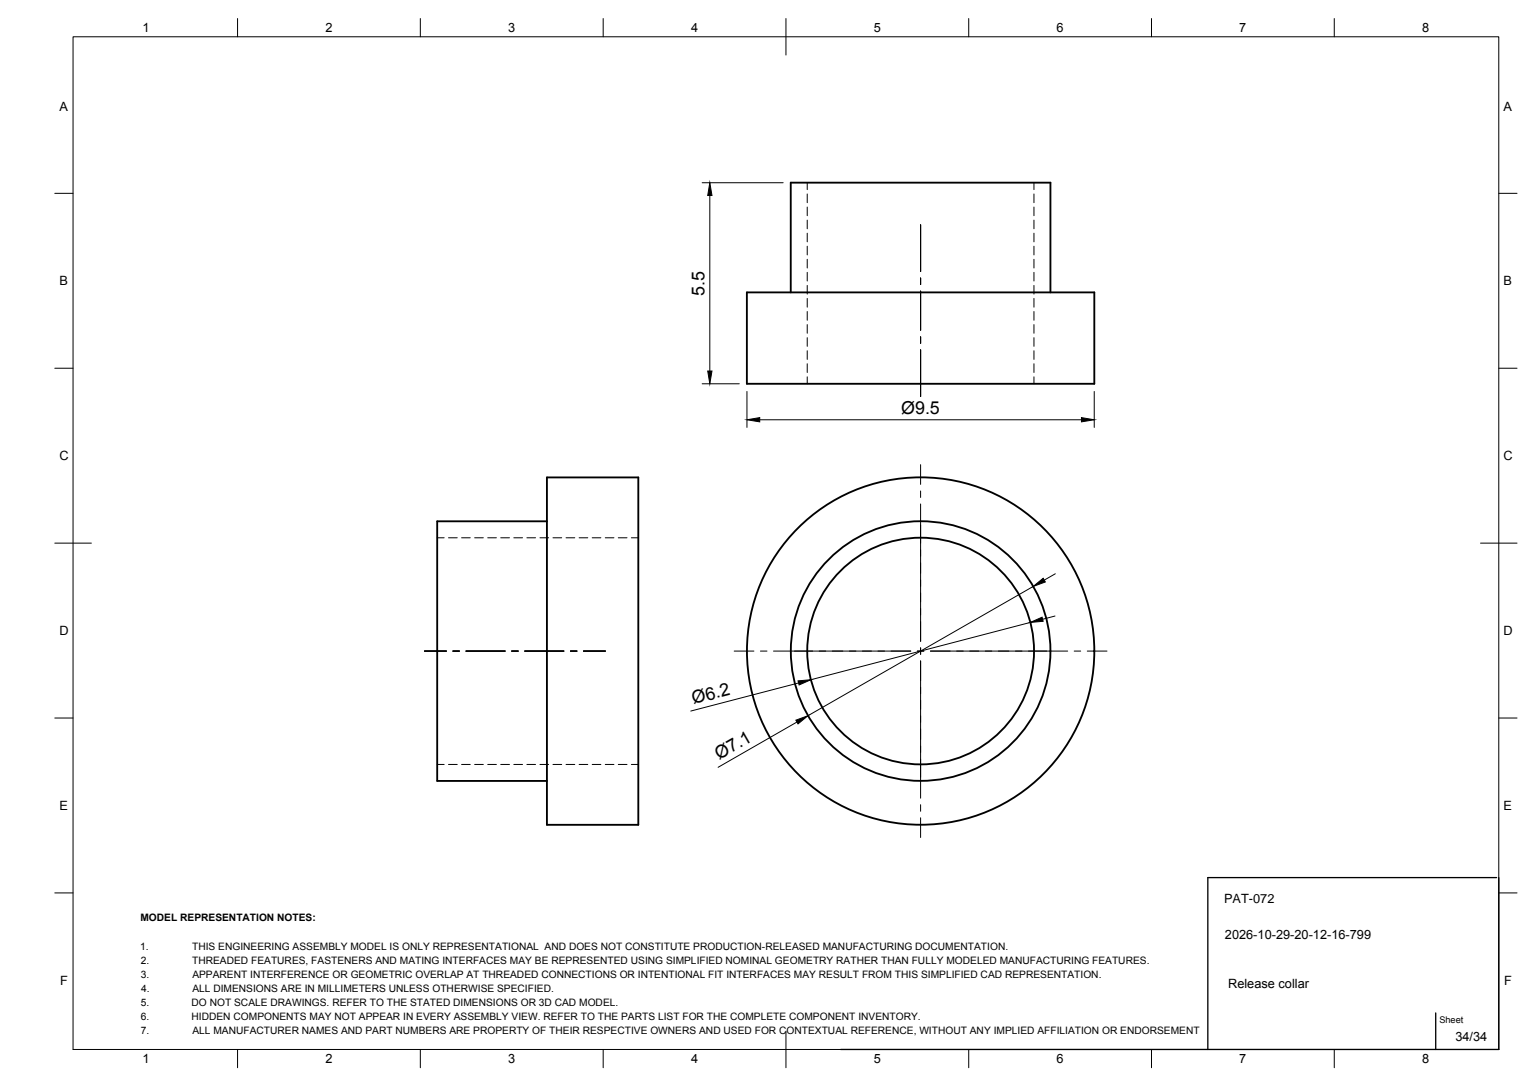
ISO-10303-21;
HEADER;
/* Generated by software containing ST-Developer
 * from STEP Tools, Inc. (www.steptools.com) 
 */

FILE_DESCRIPTION(
/* description */ ('PAT-072'),
/* implementation_level */ '2;1');

FILE_NAME(
/* name */ 'Release collar.step',
/* time_stamp */ '2026-10-29T20:11:56-07:00',
/* author */ (''),
/* organization */ (''),
/* preprocessor_version */ 'ST-DEVELOPER v20.2',
/* originating_system */ 'Autodesk Translation Framework v15.17.0.0',
/* authorisation */ '');

FILE_SCHEMA (('AUTOMOTIVE_DESIGN { 1 0 10303 214 3 1 1 }'));
ENDSEC;

DATA;
#10=MECHANICAL_DESIGN_GEOMETRIC_PRESENTATION_REPRESENTATION('',(#365),#11432);
#293=SHAPE_REPRESENTATION_RELATIONSHIP('SRR','None',#11598,#329);
#329=ADVANCED_BREP_SHAPE_REPRESENTATION('',(#400),#11429);
#365=STYLED_ITEM('',(#11833),#400);
#400=MANIFOLD_SOLID_BREP('Body1',#6101);
#562=FACE_BOUND('',#1663,.T.);
#563=FACE_BOUND('',#1666,.T.);
#564=FACE_BOUND('',#1669,.T.);
#772=PLANE('',#7147);
#773=PLANE('',#7152);
#774=PLANE('',#7156);
#1130=FACE_OUTER_BOUND('',#1662,.T.);
#1131=FACE_OUTER_BOUND('',#1664,.T.);
#1132=FACE_OUTER_BOUND('',#1665,.T.);
#1133=FACE_OUTER_BOUND('',#1667,.T.);
#1134=FACE_OUTER_BOUND('',#1668,.T.);
#1135=FACE_OUTER_BOUND('',#1670,.T.);
#1662=EDGE_LOOP('',(#5414));
#1663=EDGE_LOOP('',(#5415));
#1664=EDGE_LOOP('',(#5416,#5417,#5418,#5419));
#1665=EDGE_LOOP('',(#5420));
#1666=EDGE_LOOP('',(#5421));
#1667=EDGE_LOOP('',(#5422,#5423,#5424,#5425));
#1668=EDGE_LOOP('',(#5426));
#1669=EDGE_LOOP('',(#5427));
#1670=EDGE_LOOP('',(#5428,#5429,#5430,#5431));
#2077=LINE('',#11155,#2496);
#2078=LINE('',#11162,#2497);
#2079=LINE('',#11167,#2498);
#2496=VECTOR('',#8928,0.475);
#2497=VECTOR('',#8937,0.355);
#2498=VECTOR('',#8944,0.31);
#2814=CIRCLE('',#7148,0.475);
#2815=CIRCLE('',#7149,0.31);
#2816=CIRCLE('',#7151,0.475);
#2817=CIRCLE('',#7153,0.355);
#2818=CIRCLE('',#7155,0.355);
#2819=CIRCLE('',#7157,0.31);
#3277=VERTEX_POINT('',#11148);
#3278=VERTEX_POINT('',#11150);
#3279=VERTEX_POINT('',#11153);
#3280=VERTEX_POINT('',#11157);
#3281=VERTEX_POINT('',#11160);
#3282=VERTEX_POINT('',#11164);
#3996=EDGE_CURVE('',#3277,#3277,#2814,.T.);
#3997=EDGE_CURVE('',#3278,#3278,#2815,.T.);
#3998=EDGE_CURVE('',#3279,#3279,#2816,.T.);
#3999=EDGE_CURVE('',#3279,#3277,#2077,.T.);
#4000=EDGE_CURVE('',#3280,#3280,#2817,.T.);
#4001=EDGE_CURVE('',#3281,#3281,#2818,.T.);
#4002=EDGE_CURVE('',#3281,#3280,#2078,.T.);
#4003=EDGE_CURVE('',#3282,#3282,#2819,.T.);
#4004=EDGE_CURVE('',#3282,#3278,#2079,.T.);
#5414=ORIENTED_EDGE('',*,*,#3996,.F.);
#5415=ORIENTED_EDGE('',*,*,#3997,.T.);
#5416=ORIENTED_EDGE('',*,*,#3998,.F.);
#5417=ORIENTED_EDGE('',*,*,#3999,.T.);
#5418=ORIENTED_EDGE('',*,*,#3996,.T.);
#5419=ORIENTED_EDGE('',*,*,#3999,.F.);
#5420=ORIENTED_EDGE('',*,*,#3998,.T.);
#5421=ORIENTED_EDGE('',*,*,#4000,.F.);
#5422=ORIENTED_EDGE('',*,*,#4001,.F.);
#5423=ORIENTED_EDGE('',*,*,#4002,.T.);
#5424=ORIENTED_EDGE('',*,*,#4000,.T.);
#5425=ORIENTED_EDGE('',*,*,#4002,.F.);
#5426=ORIENTED_EDGE('',*,*,#4001,.T.);
#5427=ORIENTED_EDGE('',*,*,#4003,.F.);
#5428=ORIENTED_EDGE('',*,*,#4003,.T.);
#5429=ORIENTED_EDGE('',*,*,#4004,.T.);
#5430=ORIENTED_EDGE('',*,*,#3997,.F.);
#5431=ORIENTED_EDGE('',*,*,#4004,.F.);
#5687=CYLINDRICAL_SURFACE('',#7150,0.475);
#5688=CYLINDRICAL_SURFACE('',#7154,0.355);
#5689=CYLINDRICAL_SURFACE('',#7158,0.31);
#6029=ADVANCED_FACE('',(#1130,#562),#772,.T.);
#6030=ADVANCED_FACE('',(#1131),#5687,.T.);
#6031=ADVANCED_FACE('',(#1132,#563),#773,.T.);
#6032=ADVANCED_FACE('',(#1133),#5688,.T.);
#6033=ADVANCED_FACE('',(#1134,#564),#774,.T.);
#6034=ADVANCED_FACE('',(#1135),#5689,.F.);
#6101=CLOSED_SHELL('',(#6029,#6030,#6031,#6032,#6033,#6034));
#7146=AXIS2_PLACEMENT_3D('',#11146,#8916,#8917);
#7147=AXIS2_PLACEMENT_3D('',#11147,#8918,#8919);
#7148=AXIS2_PLACEMENT_3D('',#11149,#8920,#8921);
#7149=AXIS2_PLACEMENT_3D('',#11151,#8922,#8923);
#7150=AXIS2_PLACEMENT_3D('',#11152,#8924,#8925);
#7151=AXIS2_PLACEMENT_3D('',#11154,#8926,#8927);
#7152=AXIS2_PLACEMENT_3D('',#11156,#8929,#8930);
#7153=AXIS2_PLACEMENT_3D('',#11158,#8931,#8932);
#7154=AXIS2_PLACEMENT_3D('',#11159,#8933,#8934);
#7155=AXIS2_PLACEMENT_3D('',#11161,#8935,#8936);
#7156=AXIS2_PLACEMENT_3D('',#11163,#8938,#8939);
#7157=AXIS2_PLACEMENT_3D('',#11165,#8940,#8941);
#7158=AXIS2_PLACEMENT_3D('',#11166,#8942,#8943);
#8916=DIRECTION('axis',(0.,0.,1.));
#8917=DIRECTION('refdir',(1.,0.,0.));
#8918=DIRECTION('center_axis',(0.,1.,0.));
#8919=DIRECTION('ref_axis',(0.,0.,1.));
#8920=DIRECTION('center_axis',(0.,-1.,0.));
#8921=DIRECTION('ref_axis',(1.,0.,0.));
#8922=DIRECTION('center_axis',(0.,-1.,0.));
#8923=DIRECTION('ref_axis',(1.,0.,0.));
#8924=DIRECTION('center_axis',(0.,-1.,0.));
#8925=DIRECTION('ref_axis',(1.,0.,0.));
#8926=DIRECTION('center_axis',(0.,-1.,0.));
#8927=DIRECTION('ref_axis',(1.,0.,0.));
#8928=DIRECTION('',(0.,1.,0.));
#8929=DIRECTION('center_axis',(0.,-1.,0.));
#8930=DIRECTION('ref_axis',(0.,0.,-1.));
#8931=DIRECTION('center_axis',(0.,-1.,0.));
#8932=DIRECTION('ref_axis',(1.,0.,0.));
#8933=DIRECTION('center_axis',(0.,-1.,0.));
#8934=DIRECTION('ref_axis',(1.,0.,0.));
#8935=DIRECTION('center_axis',(0.,-1.,0.));
#8936=DIRECTION('ref_axis',(1.,0.,0.));
#8937=DIRECTION('',(0.,1.,0.));
#8938=DIRECTION('center_axis',(0.,-1.,0.));
#8939=DIRECTION('ref_axis',(0.,0.,-1.));
#8940=DIRECTION('center_axis',(0.,-1.,0.));
#8941=DIRECTION('ref_axis',(1.,0.,0.));
#8942=DIRECTION('center_axis',(0.,-1.,0.));
#8943=DIRECTION('ref_axis',(1.,0.,0.));
#8944=DIRECTION('',(0.,1.,0.));
#11146=CARTESIAN_POINT('',(0.,0.,0.));
#11147=CARTESIAN_POINT('Origin',(0.475,1.95,0.));
#11148=CARTESIAN_POINT('',(-0.475,1.95,-5.81707229594993E-17));
#11149=CARTESIAN_POINT('Origin',(0.,1.95,0.));
#11150=CARTESIAN_POINT('',(-0.31,1.95,-3.7964050773568E-17));
#11151=CARTESIAN_POINT('Origin',(0.,1.95,0.));
#11152=CARTESIAN_POINT('Origin',(0.,1.825,0.));
#11153=CARTESIAN_POINT('',(-0.475,1.7,-5.81707229594993E-17));
#11154=CARTESIAN_POINT('Origin',(0.,1.7,0.));
#11155=CARTESIAN_POINT('',(-0.475,1.825,-5.81707229594993E-17));
#11156=CARTESIAN_POINT('Origin',(0.355,1.7,0.));
#11157=CARTESIAN_POINT('',(-0.355,1.7,-4.3474961369731E-17));
#11158=CARTESIAN_POINT('Origin',(0.,1.7,0.));
#11159=CARTESIAN_POINT('Origin',(0.,1.55,0.));
#11160=CARTESIAN_POINT('',(-0.355,1.4,-4.3474961369731E-17));
#11161=CARTESIAN_POINT('Origin',(0.,1.4,0.));
#11162=CARTESIAN_POINT('',(-0.355,1.55,-4.3474961369731E-17));
#11163=CARTESIAN_POINT('Origin',(0.31,1.4,0.));
#11164=CARTESIAN_POINT('',(-0.31,1.4,-3.7964050773568E-17));
#11165=CARTESIAN_POINT('Origin',(0.,1.4,0.));
#11166=CARTESIAN_POINT('Origin',(0.,1.675,0.));
#11167=CARTESIAN_POINT('',(-0.31,1.675,-3.7964050773568E-17));
#11390=UNCERTAINTY_MEASURE_WITH_UNIT(LENGTH_MEASURE(0.001),#11433,
'DISTANCE_ACCURACY_VALUE',
'Maximum model space distance between geometric entities at asserted c
onnectivities');
#11393=UNCERTAINTY_MEASURE_WITH_UNIT(LENGTH_MEASURE(0.001),#11433,
'DISTANCE_ACCURACY_VALUE',
'Maximum model space distance between geometric entities at asserted c
onnectivities');
#11429=(
GEOMETRIC_REPRESENTATION_CONTEXT(3)
GLOBAL_UNCERTAINTY_ASSIGNED_CONTEXT((#11390))
GLOBAL_UNIT_ASSIGNED_CONTEXT((#11433,#11435,#11436))
REPRESENTATION_CONTEXT('','3D')
);
#11432=(
GEOMETRIC_REPRESENTATION_CONTEXT(3)
GLOBAL_UNCERTAINTY_ASSIGNED_CONTEXT((#11393))
GLOBAL_UNIT_ASSIGNED_CONTEXT((#11433,#11435,#11436))
REPRESENTATION_CONTEXT('','3D')
);
#11433=(
LENGTH_UNIT()
NAMED_UNIT(*)
SI_UNIT(.CENTI.,.METRE.)
);
#11435=(
NAMED_UNIT(*)
PLANE_ANGLE_UNIT()
SI_UNIT($,.RADIAN.)
);
#11436=(
NAMED_UNIT(*)
SI_UNIT($,.STERADIAN.)
SOLID_ANGLE_UNIT()
);
#11472=SHAPE_DEFINITION_REPRESENTATION(#11510,#11598);
#11510=PRODUCT_DEFINITION_SHAPE('',$,#11637);
#11598=SHAPE_REPRESENTATION('',(#7146),#11429);
#11601=PRODUCT_DEFINITION_CONTEXT('part definition',#11717,'design');
#11637=PRODUCT_DEFINITION('Release collar','Release collar',#11675,
#11601);
#11675=PRODUCT_DEFINITION_FORMATION('',$,#11754);
#11717=APPLICATION_CONTEXT(
'Core Data for Automotive Mechanical Design Process');
#11718=PRODUCT_CONTEXT('part definition',#11717,'mechanical');
#11754=PRODUCT('Release collar','Release collar',
'Release collar',(#11718));
#11827=COLOUR_RGB('Off White',0.89,0.88,0.83);
#11828=FILL_AREA_STYLE_COLOUR('',#11827);
#11829=FILL_AREA_STYLE('',(#11828));
#11830=SURFACE_STYLE_FILL_AREA(#11829);
#11831=SURFACE_SIDE_STYLE('',(#11830));
#11832=SURFACE_STYLE_USAGE(.BOTH.,#11831);
#11833=PRESENTATION_STYLE_ASSIGNMENT((#11832));
ENDSEC;
END-ISO-10303-21;
